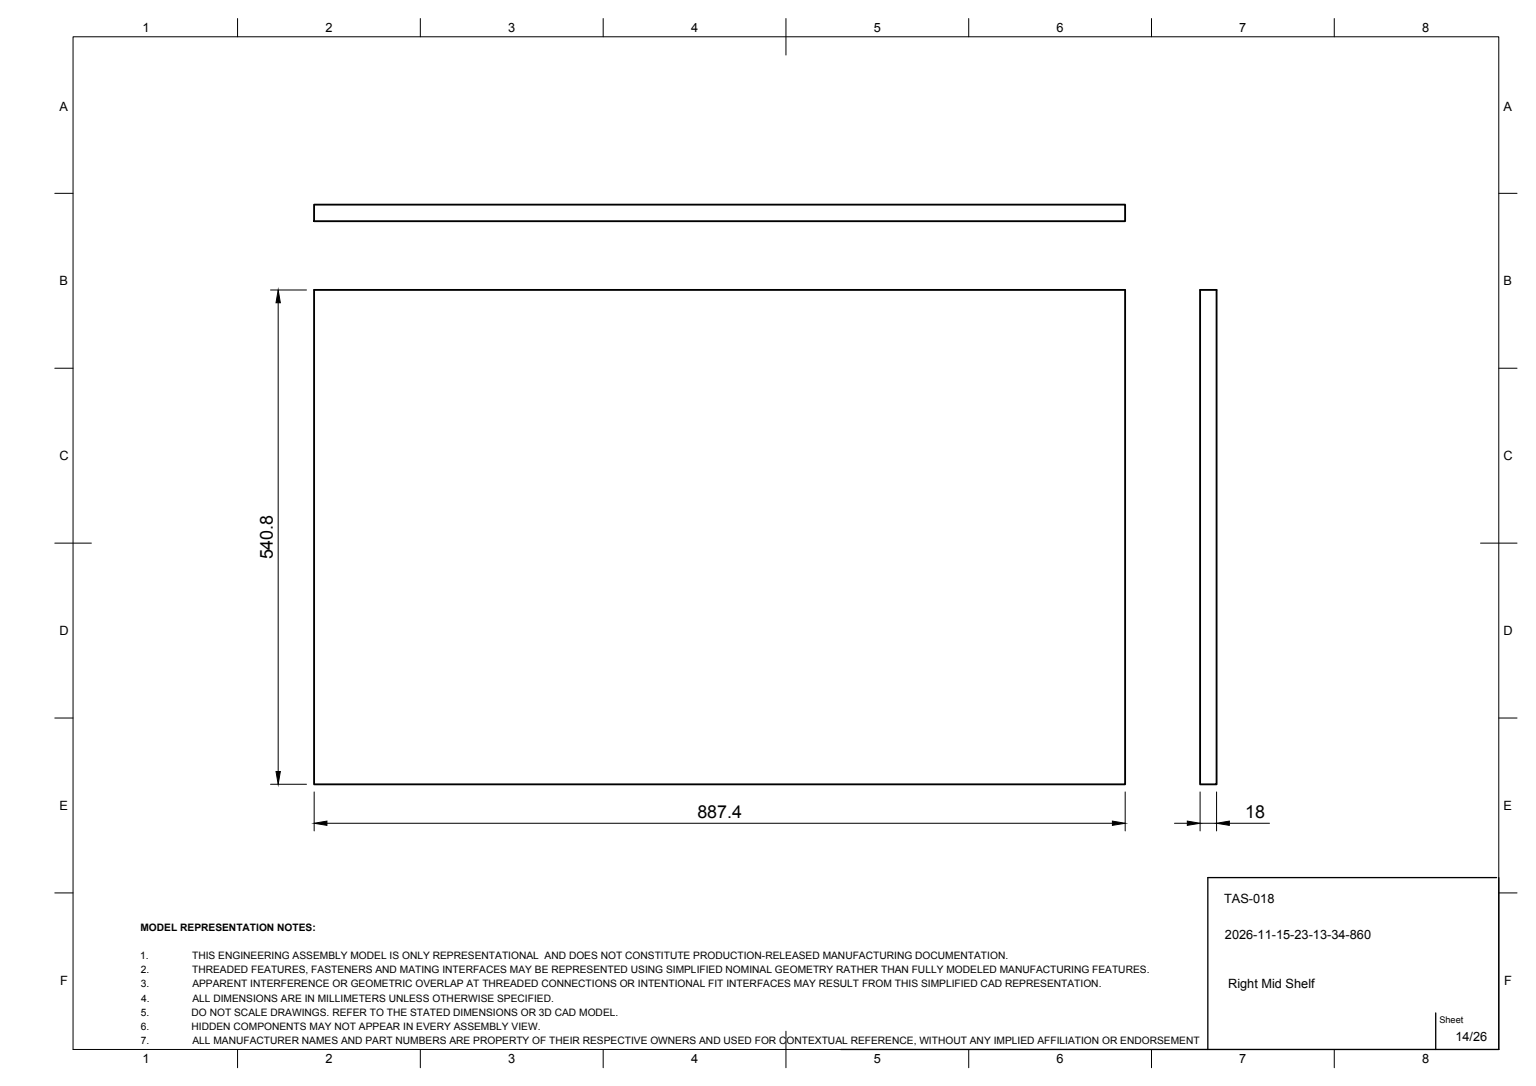
ISO-10303-21;
HEADER;
/* Generated by software containing ST-Developer
 * from STEP Tools, Inc. (www.steptools.com) 
 */

FILE_DESCRIPTION(
/* description */ (''),
/* implementation_level */ '2;1');

FILE_NAME(
/* name */ 'Right Mid Shelf.step',
/* time_stamp */ '2026-11-15T15:17:57-08:00',
/* author */ (''),
/* organization */ (''),
/* preprocessor_version */ 'ST-DEVELOPER v20.2',
/* originating_system */ 'Autodesk Translation Framework v15.17.0.0',
/* authorisation */ '');

FILE_SCHEMA (('AUTOMOTIVE_DESIGN { 1 0 10303 214 3 1 1 }'));
ENDSEC;

DATA;
#10=MECHANICAL_DESIGN_GEOMETRIC_PRESENTATION_REPRESENTATION('',(#189),#3723);
#141=SHAPE_REPRESENTATION_RELATIONSHIP('SRR','None',#3822,#165);
#165=ADVANCED_BREP_SHAPE_REPRESENTATION('',(#213),#3711);
#189=STYLED_ITEM('',(#3947),#213);
#213=MANIFOLD_SOLID_BREP('Body1',#2037);
#291=FACE_OUTER_BOUND('',#417,.T.);
#292=FACE_OUTER_BOUND('',#418,.T.);
#293=FACE_OUTER_BOUND('',#419,.T.);
#294=FACE_OUTER_BOUND('',#420,.T.);
#295=FACE_OUTER_BOUND('',#421,.T.);
#296=FACE_OUTER_BOUND('',#422,.T.);
#417=EDGE_LOOP('',(#1563,#1564,#1565,#1566));
#418=EDGE_LOOP('',(#1567,#1568,#1569,#1570));
#419=EDGE_LOOP('',(#1571,#1572,#1573,#1574));
#420=EDGE_LOOP('',(#1575,#1576,#1577,#1578));
#421=EDGE_LOOP('',(#1579,#1580,#1581,#1582));
#422=EDGE_LOOP('',(#1583,#1584,#1585,#1586));
#599=LINE('',#3398,#821);
#600=LINE('',#3400,#822);
#601=LINE('',#3402,#823);
#602=LINE('',#3403,#824);
#603=LINE('',#3407,#825);
#604=LINE('',#3409,#826);
#605=LINE('',#3411,#827);
#606=LINE('',#3412,#828);
#607=LINE('',#3414,#829);
#608=LINE('',#3415,#830);
#609=LINE('',#3417,#831);
#610=LINE('',#3419,#832);
#821=VECTOR('',#2799,34.9370078740157);
#822=VECTOR('',#2800,0.708661417322833);
#823=VECTOR('',#2801,34.9370078740157);
#824=VECTOR('',#2802,0.708661417322833);
#825=VECTOR('',#2805,0.708661417322833);
#826=VECTOR('',#2806,34.9370078740157);
#827=VECTOR('',#2807,0.708661417322833);
#828=VECTOR('',#2808,34.9370078740157);
#829=VECTOR('',#2811,21.2913385826772);
#830=VECTOR('',#2812,21.2913385826772);
#831=VECTOR('',#2815,21.2913385826772);
#832=VECTOR('',#2818,21.2913385826772);
#1005=VERTEX_POINT('',#3396);
#1006=VERTEX_POINT('',#3397);
#1007=VERTEX_POINT('',#3399);
#1008=VERTEX_POINT('',#3401);
#1009=VERTEX_POINT('',#3405);
#1010=VERTEX_POINT('',#3406);
#1011=VERTEX_POINT('',#3408);
#1012=VERTEX_POINT('',#3410);
#1203=EDGE_CURVE('',#1005,#1006,#599,.T.);
#1204=EDGE_CURVE('',#1005,#1007,#600,.T.);
#1205=EDGE_CURVE('',#1007,#1008,#601,.T.);
#1206=EDGE_CURVE('',#1006,#1008,#602,.T.);
#1207=EDGE_CURVE('',#1009,#1010,#603,.T.);
#1208=EDGE_CURVE('',#1009,#1011,#604,.T.);
#1209=EDGE_CURVE('',#1011,#1012,#605,.T.);
#1210=EDGE_CURVE('',#1010,#1012,#606,.T.);
#1211=EDGE_CURVE('',#1005,#1009,#607,.T.);
#1212=EDGE_CURVE('',#1006,#1011,#608,.T.);
#1213=EDGE_CURVE('',#1008,#1012,#609,.T.);
#1214=EDGE_CURVE('',#1007,#1010,#610,.T.);
#1563=ORIENTED_EDGE('',*,*,#1203,.F.);
#1564=ORIENTED_EDGE('',*,*,#1204,.T.);
#1565=ORIENTED_EDGE('',*,*,#1205,.T.);
#1566=ORIENTED_EDGE('',*,*,#1206,.F.);
#1567=ORIENTED_EDGE('',*,*,#1207,.F.);
#1568=ORIENTED_EDGE('',*,*,#1208,.T.);
#1569=ORIENTED_EDGE('',*,*,#1209,.T.);
#1570=ORIENTED_EDGE('',*,*,#1210,.F.);
#1571=ORIENTED_EDGE('',*,*,#1211,.F.);
#1572=ORIENTED_EDGE('',*,*,#1203,.T.);
#1573=ORIENTED_EDGE('',*,*,#1212,.T.);
#1574=ORIENTED_EDGE('',*,*,#1208,.F.);
#1575=ORIENTED_EDGE('',*,*,#1212,.F.);
#1576=ORIENTED_EDGE('',*,*,#1206,.T.);
#1577=ORIENTED_EDGE('',*,*,#1213,.T.);
#1578=ORIENTED_EDGE('',*,*,#1209,.F.);
#1579=ORIENTED_EDGE('',*,*,#1205,.F.);
#1580=ORIENTED_EDGE('',*,*,#1214,.T.);
#1581=ORIENTED_EDGE('',*,*,#1210,.T.);
#1582=ORIENTED_EDGE('',*,*,#1213,.F.);
#1583=ORIENTED_EDGE('',*,*,#1204,.F.);
#1584=ORIENTED_EDGE('',*,*,#1211,.T.);
#1585=ORIENTED_EDGE('',*,*,#1207,.T.);
#1586=ORIENTED_EDGE('',*,*,#1214,.F.);
#1843=PLANE('',#2400);
#1844=PLANE('',#2401);
#1845=PLANE('',#2402);
#1846=PLANE('',#2403);
#1847=PLANE('',#2404);
#1848=PLANE('',#2405);
#1965=ADVANCED_FACE('',(#291),#1843,.T.);
#1966=ADVANCED_FACE('',(#292),#1844,.F.);
#1967=ADVANCED_FACE('',(#293),#1845,.T.);
#1968=ADVANCED_FACE('',(#294),#1846,.T.);
#1969=ADVANCED_FACE('',(#295),#1847,.F.);
#1970=ADVANCED_FACE('',(#296),#1848,.F.);
#2037=CLOSED_SHELL('',(#1965,#1966,#1967,#1968,#1969,#1970));
#2399=AXIS2_PLACEMENT_3D('',#3394,#2795,#2796);
#2400=AXIS2_PLACEMENT_3D('',#3395,#2797,#2798);
#2401=AXIS2_PLACEMENT_3D('',#3404,#2803,#2804);
#2402=AXIS2_PLACEMENT_3D('',#3413,#2809,#2810);
#2403=AXIS2_PLACEMENT_3D('',#3416,#2813,#2814);
#2404=AXIS2_PLACEMENT_3D('',#3418,#2816,#2817);
#2405=AXIS2_PLACEMENT_3D('',#3420,#2819,#2820);
#2795=DIRECTION('axis',(0.,0.,1.));
#2796=DIRECTION('refdir',(1.,0.,0.));
#2797=DIRECTION('center_axis',(0.,0.,1.));
#2798=DIRECTION('ref_axis',(1.,0.,0.));
#2799=DIRECTION('',(1.,0.,0.));
#2800=DIRECTION('',(0.,-1.,0.));
#2801=DIRECTION('',(1.,0.,0.));
#2802=DIRECTION('',(0.,-1.,0.));
#2803=DIRECTION('center_axis',(0.,0.,1.));
#2804=DIRECTION('ref_axis',(1.,0.,0.));
#2805=DIRECTION('',(0.,-1.,0.));
#2806=DIRECTION('',(1.,0.,0.));
#2807=DIRECTION('',(0.,-1.,0.));
#2808=DIRECTION('',(1.,0.,0.));
#2809=DIRECTION('center_axis',(0.,1.,0.));
#2810=DIRECTION('ref_axis',(0.,0.,1.));
#2811=DIRECTION('',(0.,0.,-1.));
#2812=DIRECTION('',(0.,0.,-1.));
#2813=DIRECTION('center_axis',(1.,0.,0.));
#2814=DIRECTION('ref_axis',(0.,0.,-1.));
#2815=DIRECTION('',(0.,0.,-1.));
#2816=DIRECTION('center_axis',(0.,1.,0.));
#2817=DIRECTION('ref_axis',(0.,0.,1.));
#2818=DIRECTION('',(0.,0.,-1.));
#2819=DIRECTION('center_axis',(1.,0.,0.));
#2820=DIRECTION('ref_axis',(0.,0.,-1.));
#3394=CARTESIAN_POINT('',(0.,0.,0.));
#3395=CARTESIAN_POINT('Origin',(0.,0.,22.));
#3396=CARTESIAN_POINT('',(0.354330708661414,30.,22.));
#3397=CARTESIAN_POINT('',(35.2913385826772,30.,22.));
#3398=CARTESIAN_POINT('',(0.354330708661414,30.,22.));
#3399=CARTESIAN_POINT('',(0.354330708661414,29.2913385826772,22.));
#3400=CARTESIAN_POINT('',(0.354330708661414,30.,22.));
#3401=CARTESIAN_POINT('',(35.2913385826772,29.2913385826772,22.));
#3402=CARTESIAN_POINT('',(0.354330708661414,29.2913385826772,22.));
#3403=CARTESIAN_POINT('',(35.2913385826772,30.,22.));
#3404=CARTESIAN_POINT('Origin',(0.,0.,0.708661417322834));
#3405=CARTESIAN_POINT('',(0.354330708661414,30.,0.708661417322834));
#3406=CARTESIAN_POINT('',(0.354330708661414,29.2913385826772,0.708661417322834));
#3407=CARTESIAN_POINT('',(0.354330708661414,30.,0.708661417322834));
#3408=CARTESIAN_POINT('',(35.2913385826772,30.,0.708661417322834));
#3409=CARTESIAN_POINT('',(0.354330708661414,30.,0.708661417322834));
#3410=CARTESIAN_POINT('',(35.2913385826772,29.2913385826772,0.708661417322834));
#3411=CARTESIAN_POINT('',(35.2913385826772,30.,0.708661417322834));
#3412=CARTESIAN_POINT('',(0.354330708661414,29.2913385826772,0.708661417322834));
#3413=CARTESIAN_POINT('Origin',(0.354330708661414,30.,56.9441943703592));
#3414=CARTESIAN_POINT('',(0.354330708661414,30.,22.));
#3415=CARTESIAN_POINT('',(35.2913385826772,30.,22.));
#3416=CARTESIAN_POINT('Origin',(35.2913385826772,30.,56.9441943703592));
#3417=CARTESIAN_POINT('',(35.2913385826772,29.2913385826772,22.));
#3418=CARTESIAN_POINT('Origin',(0.354330708661414,29.2913385826772,56.9441943703592));
#3419=CARTESIAN_POINT('',(0.354330708661414,29.2913385826772,22.));
#3420=CARTESIAN_POINT('Origin',(0.354330708661414,30.,56.9441943703592));
#3684=UNCERTAINTY_MEASURE_WITH_UNIT(LENGTH_MEASURE(0.000393700787401575),
#3725,'DISTANCE_ACCURACY_VALUE',
'Maximum model space distance between geometric entities at asserted c
onnectivities');
#3696=UNCERTAINTY_MEASURE_WITH_UNIT(LENGTH_MEASURE(0.000393700787401575),
#3725,'DISTANCE_ACCURACY_VALUE',
'Maximum model space distance between geometric entities at asserted c
onnectivities');
#3711=(
GEOMETRIC_REPRESENTATION_CONTEXT(3)
GLOBAL_UNCERTAINTY_ASSIGNED_CONTEXT((#3684))
GLOBAL_UNIT_ASSIGNED_CONTEXT((#3725,#3729,#3730))
REPRESENTATION_CONTEXT('','3D')
);
#3723=(
GEOMETRIC_REPRESENTATION_CONTEXT(3)
GLOBAL_UNCERTAINTY_ASSIGNED_CONTEXT((#3696))
GLOBAL_UNIT_ASSIGNED_CONTEXT((#3725,#3729,#3730))
REPRESENTATION_CONTEXT('','3D')
);
#3724=DIMENSIONAL_EXPONENTS(1.,0.,0.,0.,0.,0.,0.);
#3725=(
CONVERSION_BASED_UNIT('inch',#3728)
LENGTH_UNIT()
NAMED_UNIT(#3724)
);
#3726=(
LENGTH_UNIT()
NAMED_UNIT(*)
SI_UNIT(.MILLI.,.METRE.)
);
#3728=LENGTH_MEASURE_WITH_UNIT(LENGTH_MEASURE(25.4),#3726);
#3729=(
NAMED_UNIT(*)
PLANE_ANGLE_UNIT()
SI_UNIT($,.RADIAN.)
);
#3730=(
NAMED_UNIT(*)
SI_UNIT($,.STERADIAN.)
SOLID_ANGLE_UNIT()
);
#3745=SHAPE_DEFINITION_REPRESENTATION(#3772,#3822);
#3772=PRODUCT_DEFINITION_SHAPE('',$,#3849);
#3822=SHAPE_REPRESENTATION('',(#2399),#3711);
#3834=PRODUCT_DEFINITION_CONTEXT('part definition',#3914,'design');
#3849=PRODUCT_DEFINITION('2026-11-15-23-13-34-860','Right Mid Shelf',#3875,
#3834);
#3875=PRODUCT_DEFINITION_FORMATION('',$,#3930);
#3914=APPLICATION_CONTEXT(
'Core Data for Automotive Mechanical Design Process');
#3915=PRODUCT_CONTEXT('part definition',#3914,'mechanical');
#3930=PRODUCT('2026-11-15-23-13-34-860','Right Mid Shelf',$,(#3915));
#3947=PRESENTATION_STYLE_ASSIGNMENT((#3955));
#3955=SURFACE_STYLE_USAGE(.BOTH.,#3963);
#3963=SURFACE_SIDE_STYLE('',(#3971));
#3971=SURFACE_STYLE_FILL_AREA(#3979);
#3979=FILL_AREA_STYLE('Light Blue',(#3987));
#3987=FILL_AREA_STYLE_COLOUR('Light Blue',#3995);
#3995=COLOUR_RGB('Light Blue',0.67843137254902,0.847058823529412,0.901960784313726);
ENDSEC;
END-ISO-10303-21;
